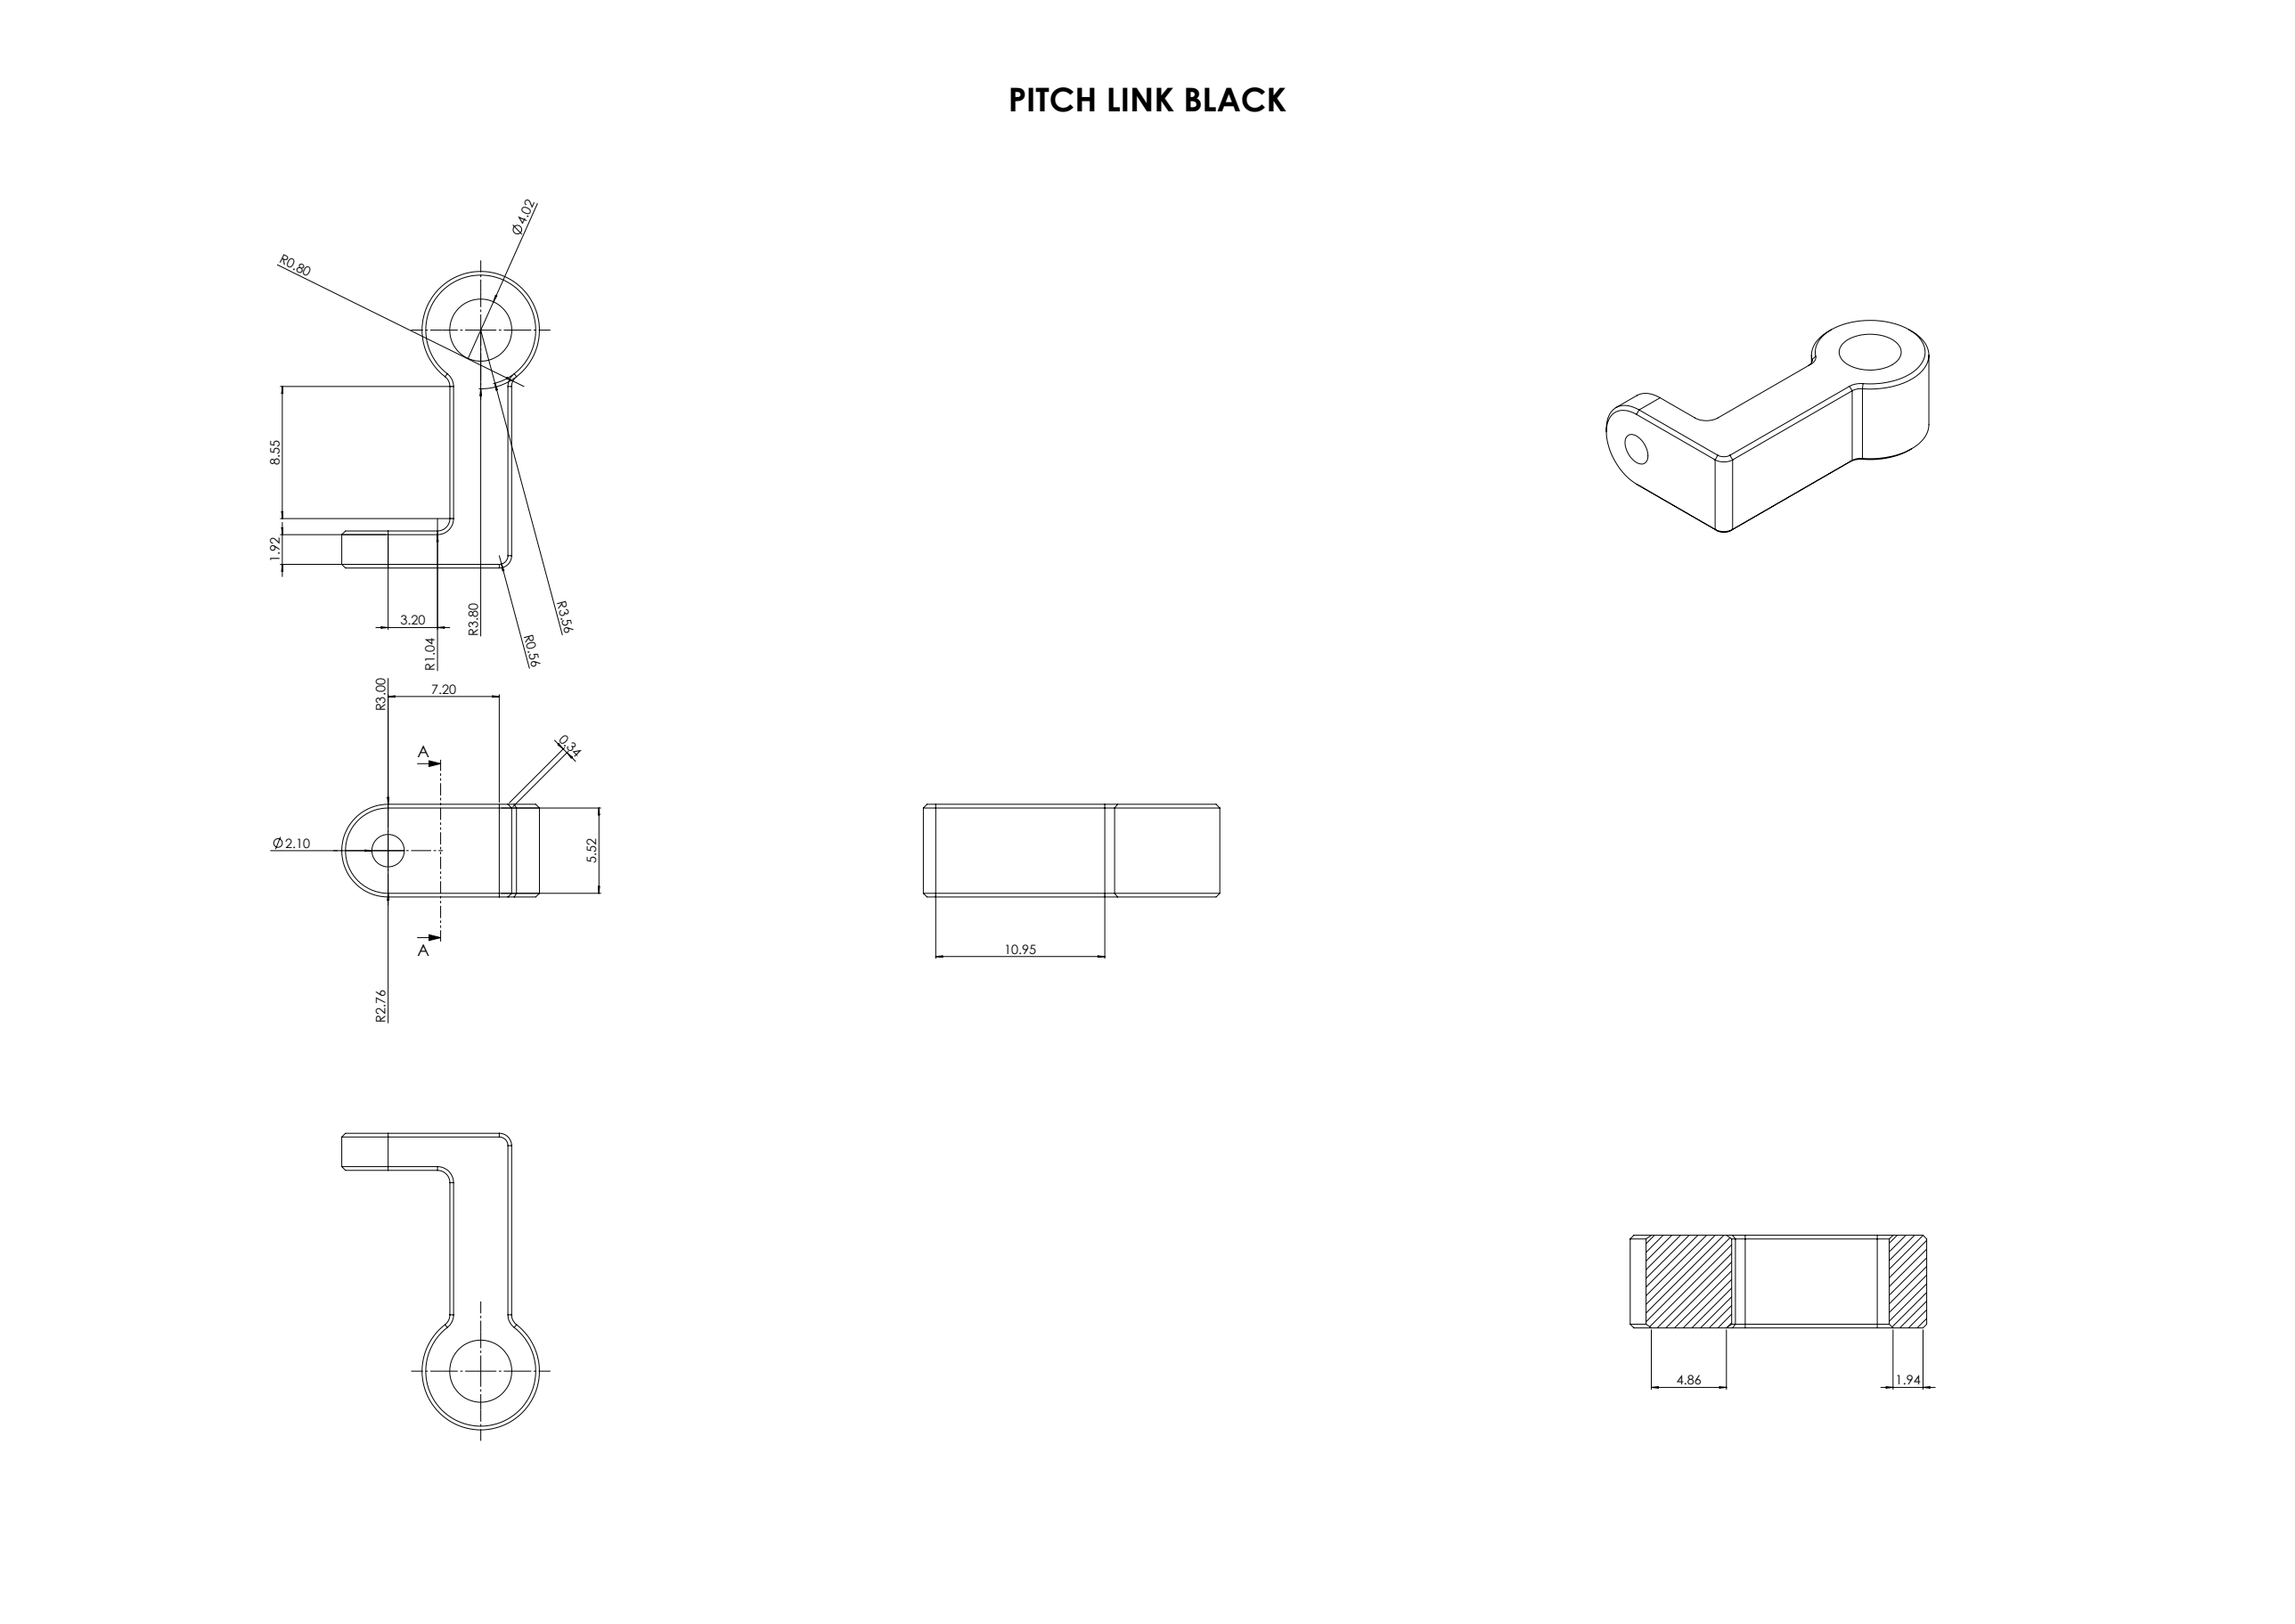
ISO-10303-21;
HEADER;
/* Generated by software containing ST-Developer
 * from STEP Tools, Inc. (www.steptools.com) 
 */

FILE_DESCRIPTION(
/* description */ (''),
/* implementation_level */ '2;1');

FILE_NAME(
/* name */ '07_Pitch_Link_Black.step',
/* time_stamp */ '2026-10-25T01:35:35-07:00',
/* author */ (''),
/* organization */ (''),
/* preprocessor_version */ 'ST-DEVELOPER v20.2',
/* originating_system */ 'Autodesk Translation Framework v15.15.0.0',
/* authorisation */ '');

FILE_SCHEMA (('AUTOMOTIVE_DESIGN { 1 0 10303 214 3 1 1 }'));
ENDSEC;

DATA;
#10=MECHANICAL_DESIGN_GEOMETRIC_PRESENTATION_REPRESENTATION('',(#268),#11430);
#244=SHAPE_REPRESENTATION_RELATIONSHIP('SRR','None',#11487,#256);
#256=ADVANCED_BREP_SHAPE_REPRESENTATION('',(#280),#11426);
#268=STYLED_ITEM('',(#11623),#280);
#280=MANIFOLD_SOLID_BREP('Body1',#4469);
#312=FACE_BOUND('',#1015,.T.);
#313=FACE_BOUND('',#1022,.T.);
#314=FACE_BOUND('',#1029,.T.);
#315=FACE_BOUND('',#1031,.T.);
#395=PLANE('',#4915);
#396=PLANE('',#4919);
#397=PLANE('',#4923);
#398=PLANE('',#4927);
#399=PLANE('',#4937);
#400=PLANE('',#4941);
#401=PLANE('',#4945);
#402=PLANE('',#4949);
#403=PLANE('',#4959);
#404=PLANE('',#4965);
#405=PLANE('',#4966);
#406=PLANE('',#4969);
#407=PLANE('',#4975);
#408=PLANE('',#4976);
#486=CYLINDRICAL_SURFACE('',#4961,0.8);
#487=CYLINDRICAL_SURFACE('',#4962,3.8);
#488=CYLINDRICAL_SURFACE('',#4963,0.8);
#489=CYLINDRICAL_SURFACE('',#4964,0.8);
#490=CYLINDRICAL_SURFACE('',#4968,3.);
#491=CYLINDRICAL_SURFACE('',#4970,0.8);
#492=CYLINDRICAL_SURFACE('',#4971,2.01);
#493=CYLINDRICAL_SURFACE('',#4973,1.05);
#698=FACE_OUTER_BOUND('',#994,.T.);
#699=FACE_OUTER_BOUND('',#995,.T.);
#700=FACE_OUTER_BOUND('',#996,.T.);
#701=FACE_OUTER_BOUND('',#997,.T.);
#702=FACE_OUTER_BOUND('',#998,.T.);
#703=FACE_OUTER_BOUND('',#999,.T.);
#704=FACE_OUTER_BOUND('',#1000,.T.);
#705=FACE_OUTER_BOUND('',#1001,.T.);
#706=FACE_OUTER_BOUND('',#1002,.T.);
#707=FACE_OUTER_BOUND('',#1003,.T.);
#708=FACE_OUTER_BOUND('',#1004,.T.);
#709=FACE_OUTER_BOUND('',#1005,.T.);
#710=FACE_OUTER_BOUND('',#1006,.T.);
#711=FACE_OUTER_BOUND('',#1007,.T.);
#712=FACE_OUTER_BOUND('',#1008,.T.);
#713=FACE_OUTER_BOUND('',#1009,.T.);
#714=FACE_OUTER_BOUND('',#1010,.T.);
#715=FACE_OUTER_BOUND('',#1011,.T.);
#716=FACE_OUTER_BOUND('',#1012,.T.);
#717=FACE_OUTER_BOUND('',#1013,.T.);
#718=FACE_OUTER_BOUND('',#1014,.T.);
#719=FACE_OUTER_BOUND('',#1016,.T.);
#720=FACE_OUTER_BOUND('',#1017,.T.);
#721=FACE_OUTER_BOUND('',#1018,.T.);
#722=FACE_OUTER_BOUND('',#1019,.T.);
#723=FACE_OUTER_BOUND('',#1020,.T.);
#724=FACE_OUTER_BOUND('',#1021,.T.);
#725=FACE_OUTER_BOUND('',#1023,.T.);
#726=FACE_OUTER_BOUND('',#1024,.T.);
#727=FACE_OUTER_BOUND('',#1025,.T.);
#728=FACE_OUTER_BOUND('',#1026,.T.);
#729=FACE_OUTER_BOUND('',#1027,.T.);
#730=FACE_OUTER_BOUND('',#1028,.T.);
#731=FACE_OUTER_BOUND('',#1030,.T.);
#994=EDGE_LOOP('',(#3675,#3676,#3677,#3678));
#995=EDGE_LOOP('',(#3679,#3680,#3681,#3682));
#996=EDGE_LOOP('',(#3683,#3684,#3685,#3686));
#997=EDGE_LOOP('',(#3687,#3688,#3689,#3690));
#998=EDGE_LOOP('',(#3691,#3692,#3693,#3694));
#999=EDGE_LOOP('',(#3695,#3696,#3697,#3698));
#1000=EDGE_LOOP('',(#3699,#3700,#3701,#3702));
#1001=EDGE_LOOP('',(#3703,#3704,#3705,#3706));
#1002=EDGE_LOOP('',(#3707,#3708,#3709,#3710));
#1003=EDGE_LOOP('',(#3711,#3712,#3713,#3714));
#1004=EDGE_LOOP('',(#3715,#3716,#3717,#3718));
#1005=EDGE_LOOP('',(#3719,#3720,#3721,#3722));
#1006=EDGE_LOOP('',(#3723,#3724,#3725,#3726));
#1007=EDGE_LOOP('',(#3727,#3728,#3729,#3730));
#1008=EDGE_LOOP('',(#3731,#3732,#3733,#3734));
#1009=EDGE_LOOP('',(#3735,#3736,#3737,#3738));
#1010=EDGE_LOOP('',(#3739,#3740,#3741,#3742));
#1011=EDGE_LOOP('',(#3743,#3744,#3745,#3746));
#1012=EDGE_LOOP('',(#3747,#3748,#3749,#3750));
#1013=EDGE_LOOP('',(#3751,#3752,#3753,#3754));
#1014=EDGE_LOOP('',(#3755,#3756,#3757,#3758));
#1015=EDGE_LOOP('',(#3759));
#1016=EDGE_LOOP('',(#3760,#3761,#3762,#3763));
#1017=EDGE_LOOP('',(#3764,#3765,#3766,#3767));
#1018=EDGE_LOOP('',(#3768,#3769,#3770,#3771));
#1019=EDGE_LOOP('',(#3772,#3773,#3774,#3775));
#1020=EDGE_LOOP('',(#3776,#3777,#3778,#3779));
#1021=EDGE_LOOP('',(#3780,#3781,#3782,#3783,#3784,#3785,#3786,#3787,#3788,
#3789));
#1022=EDGE_LOOP('',(#3790));
#1023=EDGE_LOOP('',(#3791,#3792,#3793,#3794));
#1024=EDGE_LOOP('',(#3795,#3796,#3797,#3798));
#1025=EDGE_LOOP('',(#3799,#3800,#3801,#3802));
#1026=EDGE_LOOP('',(#3803,#3804,#3805,#3806));
#1027=EDGE_LOOP('',(#3807,#3808,#3809,#3810));
#1028=EDGE_LOOP('',(#3811,#3812,#3813,#3814,#3815,#3816,#3817,#3818,#3819,
#3820));
#1029=EDGE_LOOP('',(#3821));
#1030=EDGE_LOOP('',(#3822,#3823,#3824,#3825));
#1031=EDGE_LOOP('',(#3826));
#1271=LINE('',#9219,#1561);
#1272=LINE('',#9221,#1562);
#1273=LINE('',#9223,#1563);
#1274=LINE('',#9224,#1564);
#1275=LINE('',#9229,#1565);
#1276=LINE('',#9233,#1566);
#1277=LINE('',#9235,#1567);
#1278=LINE('',#9236,#1568);
#1279=LINE('',#9241,#1569);
#1280=LINE('',#9245,#1570);
#1281=LINE('',#9247,#1571);
#1282=LINE('',#9248,#1572);
#1283=LINE('',#9253,#1573);
#1284=LINE('',#9258,#1574);
#1285=LINE('',#9259,#1575);
#1286=LINE('',#9260,#1576);
#1287=LINE('',#9265,#1577);
#1288=LINE('',#9270,#1578);
#1289=LINE('',#9277,#1579);
#1290=LINE('',#9282,#1580);
#1291=LINE('',#9283,#1581);
#1292=LINE('',#9284,#1582);
#1293=LINE('',#9289,#1583);
#1294=LINE('',#9294,#1584);
#1295=LINE('',#9295,#1585);
#1296=LINE('',#9296,#1586);
#1297=LINE('',#9300,#1587);
#1298=LINE('',#9306,#1588);
#1299=LINE('',#9307,#1589);
#1300=LINE('',#9308,#1590);
#1301=LINE('',#9313,#1591);
#1302=LINE('',#9317,#1592);
#1303=LINE('',#9319,#1593);
#1304=LINE('',#9320,#1594);
#1305=LINE('',#9325,#1595);
#1306=LINE('',#9331,#1596);
#1307=LINE('',#9337,#1597);
#1308=LINE('',#9341,#1598);
#1309=LINE('',#9342,#1599);
#1310=LINE('',#9344,#1600);
#1311=LINE('',#9346,#1601);
#1312=LINE('',#9348,#1602);
#1313=LINE('',#9351,#1603);
#1314=LINE('',#9355,#1604);
#1315=LINE('',#9357,#1605);
#1316=LINE('',#9359,#1606);
#1317=LINE('',#9362,#1607);
#1318=LINE('',#9366,#1608);
#1561=VECTOR('',#5873,10.);
#1562=VECTOR('',#5874,10.);
#1563=VECTOR('',#5875,10.);
#1564=VECTOR('',#5876,10.);
#1565=VECTOR('',#5881,10.);
#1566=VECTOR('',#5886,10.);
#1567=VECTOR('',#5887,10.);
#1568=VECTOR('',#5888,10.);
#1569=VECTOR('',#5893,10.);
#1570=VECTOR('',#5898,10.);
#1571=VECTOR('',#5899,10.);
#1572=VECTOR('',#5900,10.);
#1573=VECTOR('',#5905,10.);
#1574=VECTOR('',#5910,10.);
#1575=VECTOR('',#5911,10.);
#1576=VECTOR('',#5912,10.);
#1577=VECTOR('',#5917,10.);
#1578=VECTOR('',#5922,10.);
#1579=VECTOR('',#5931,10.);
#1580=VECTOR('',#5936,10.);
#1581=VECTOR('',#5937,10.);
#1582=VECTOR('',#5938,10.);
#1583=VECTOR('',#5943,10.);
#1584=VECTOR('',#5948,10.);
#1585=VECTOR('',#5949,10.);
#1586=VECTOR('',#5950,10.);
#1587=VECTOR('',#5953,10.);
#1588=VECTOR('',#5960,10.);
#1589=VECTOR('',#5961,10.);
#1590=VECTOR('',#5962,10.);
#1591=VECTOR('',#5967,10.);
#1592=VECTOR('',#5972,10.);
#1593=VECTOR('',#5973,10.);
#1594=VECTOR('',#5974,10.);
#1595=VECTOR('',#5979,10.);
#1596=VECTOR('',#5986,10.);
#1597=VECTOR('',#5997,10.);
#1598=VECTOR('',#6002,10.);
#1599=VECTOR('',#6003,10.);
#1600=VECTOR('',#6006,10.);
#1601=VECTOR('',#6009,10.);
#1602=VECTOR('',#6012,10.);
#1603=VECTOR('',#6017,10.);
#1604=VECTOR('',#6022,10.);
#1605=VECTOR('',#6025,10.);
#1606=VECTOR('',#6028,10.);
#1607=VECTOR('',#6031,2.01);
#1608=VECTOR('',#6036,1.05);
#1812=CIRCLE('',#4917,0.8);
#1813=CIRCLE('',#4918,0.56);
#1814=CIRCLE('',#4921,2.76);
#1815=CIRCLE('',#4922,3.);
#1816=CIRCLE('',#4925,0.8);
#1817=CIRCLE('',#4926,0.56);
#1818=CIRCLE('',#4929,0.8);
#1819=CIRCLE('',#4930,1.04);
#1820=CIRCLE('',#4932,3.56);
#1821=CIRCLE('',#4933,3.8);
#1822=CIRCLE('',#4935,0.8);
#1823=CIRCLE('',#4936,1.04);
#1824=CIRCLE('',#4939,0.8);
#1825=CIRCLE('',#4940,1.04);
#1826=CIRCLE('',#4943,3.);
#1827=CIRCLE('',#4944,2.76);
#1828=CIRCLE('',#4947,0.8);
#1829=CIRCLE('',#4948,1.04);
#1830=CIRCLE('',#4951,0.8);
#1831=CIRCLE('',#4952,1.04);
#1832=CIRCLE('',#4954,3.8);
#1833=CIRCLE('',#4955,3.56);
#1834=CIRCLE('',#4957,0.8);
#1835=CIRCLE('',#4958,1.04);
#1836=CIRCLE('',#4960,1.05);
#1837=CIRCLE('',#4967,2.01);
#1838=CIRCLE('',#4972,2.01);
#1839=CIRCLE('',#4974,1.05);
#2115=VERTEX_POINT('',#9217);
#2116=VERTEX_POINT('',#9218);
#2117=VERTEX_POINT('',#9220);
#2118=VERTEX_POINT('',#9222);
#2119=VERTEX_POINT('',#9226);
#2120=VERTEX_POINT('',#9228);
#2121=VERTEX_POINT('',#9232);
#2122=VERTEX_POINT('',#9234);
#2123=VERTEX_POINT('',#9238);
#2124=VERTEX_POINT('',#9240);
#2125=VERTEX_POINT('',#9244);
#2126=VERTEX_POINT('',#9246);
#2127=VERTEX_POINT('',#9250);
#2128=VERTEX_POINT('',#9252);
#2129=VERTEX_POINT('',#9256);
#2130=VERTEX_POINT('',#9257);
#2131=VERTEX_POINT('',#9262);
#2132=VERTEX_POINT('',#9264);
#2133=VERTEX_POINT('',#9268);
#2134=VERTEX_POINT('',#9269);
#2135=VERTEX_POINT('',#9274);
#2136=VERTEX_POINT('',#9276);
#2137=VERTEX_POINT('',#9280);
#2138=VERTEX_POINT('',#9281);
#2139=VERTEX_POINT('',#9286);
#2140=VERTEX_POINT('',#9288);
#2141=VERTEX_POINT('',#9292);
#2142=VERTEX_POINT('',#9293);
#2143=VERTEX_POINT('',#9298);
#2144=VERTEX_POINT('',#9299);
#2145=VERTEX_POINT('',#9304);
#2146=VERTEX_POINT('',#9305);
#2147=VERTEX_POINT('',#9310);
#2148=VERTEX_POINT('',#9312);
#2149=VERTEX_POINT('',#9316);
#2150=VERTEX_POINT('',#9318);
#2151=VERTEX_POINT('',#9322);
#2152=VERTEX_POINT('',#9324);
#2153=VERTEX_POINT('',#9328);
#2154=VERTEX_POINT('',#9330);
#2155=VERTEX_POINT('',#9338);
#2156=VERTEX_POINT('',#9352);
#2157=VERTEX_POINT('',#9361);
#2158=VERTEX_POINT('',#9365);
#2655=EDGE_CURVE('',#2115,#2116,#1271,.T.);
#2656=EDGE_CURVE('',#2116,#2117,#1272,.T.);
#2657=EDGE_CURVE('',#2117,#2118,#1273,.T.);
#2658=EDGE_CURVE('',#2118,#2115,#1274,.T.);
#2659=EDGE_CURVE('',#2115,#2119,#1812,.T.);
#2660=EDGE_CURVE('',#2119,#2120,#1275,.T.);
#2661=EDGE_CURVE('',#2120,#2116,#1813,.T.);
#2662=EDGE_CURVE('',#2119,#2121,#1276,.T.);
#2663=EDGE_CURVE('',#2121,#2122,#1277,.T.);
#2664=EDGE_CURVE('',#2122,#2120,#1278,.T.);
#2665=EDGE_CURVE('',#2121,#2123,#1814,.T.);
#2666=EDGE_CURVE('',#2123,#2124,#1279,.T.);
#2667=EDGE_CURVE('',#2124,#2122,#1815,.T.);
#2668=EDGE_CURVE('',#2123,#2125,#1280,.T.);
#2669=EDGE_CURVE('',#2125,#2126,#1281,.T.);
#2670=EDGE_CURVE('',#2126,#2124,#1282,.T.);
#2671=EDGE_CURVE('',#2125,#2127,#1816,.T.);
#2672=EDGE_CURVE('',#2127,#2128,#1283,.T.);
#2673=EDGE_CURVE('',#2128,#2126,#1817,.T.);
#2674=EDGE_CURVE('',#2129,#2130,#1284,.T.);
#2675=EDGE_CURVE('',#2130,#2128,#1285,.T.);
#2676=EDGE_CURVE('',#2127,#2129,#1286,.T.);
#2677=EDGE_CURVE('',#2129,#2131,#1818,.T.);
#2678=EDGE_CURVE('',#2131,#2132,#1287,.T.);
#2679=EDGE_CURVE('',#2132,#2130,#1819,.T.);
#2680=EDGE_CURVE('',#2133,#2134,#1288,.T.);
#2681=EDGE_CURVE('',#2134,#2132,#1820,.T.);
#2682=EDGE_CURVE('',#2131,#2133,#1821,.T.);
#2683=EDGE_CURVE('',#2133,#2135,#1822,.T.);
#2684=EDGE_CURVE('',#2135,#2136,#1289,.T.);
#2685=EDGE_CURVE('',#2136,#2134,#1823,.T.);
#2686=EDGE_CURVE('',#2137,#2138,#1290,.T.);
#2687=EDGE_CURVE('',#2138,#2136,#1291,.T.);
#2688=EDGE_CURVE('',#2135,#2137,#1292,.T.);
#2689=EDGE_CURVE('',#2137,#2139,#1824,.T.);
#2690=EDGE_CURVE('',#2139,#2140,#1293,.T.);
#2691=EDGE_CURVE('',#2140,#2138,#1825,.T.);
#2692=EDGE_CURVE('',#2141,#2142,#1294,.T.);
#2693=EDGE_CURVE('',#2142,#2140,#1295,.T.);
#2694=EDGE_CURVE('',#2139,#2141,#1296,.T.);
#2695=EDGE_CURVE('',#2143,#2144,#1297,.T.);
#2696=EDGE_CURVE('',#2144,#2142,#1826,.T.);
#2697=EDGE_CURVE('',#2141,#2143,#1827,.T.);
#2698=EDGE_CURVE('',#2145,#2146,#1298,.T.);
#2699=EDGE_CURVE('',#2146,#2144,#1299,.T.);
#2700=EDGE_CURVE('',#2143,#2145,#1300,.T.);
#2701=EDGE_CURVE('',#2145,#2147,#1828,.T.);
#2702=EDGE_CURVE('',#2147,#2148,#1301,.T.);
#2703=EDGE_CURVE('',#2148,#2146,#1829,.T.);
#2704=EDGE_CURVE('',#2147,#2149,#1302,.T.);
#2705=EDGE_CURVE('',#2149,#2150,#1303,.T.);
#2706=EDGE_CURVE('',#2150,#2148,#1304,.T.);
#2707=EDGE_CURVE('',#2149,#2151,#1830,.T.);
#2708=EDGE_CURVE('',#2151,#2152,#1305,.T.);
#2709=EDGE_CURVE('',#2152,#2150,#1831,.T.);
#2710=EDGE_CURVE('',#2151,#2153,#1832,.T.);
#2711=EDGE_CURVE('',#2153,#2154,#1306,.T.);
#2712=EDGE_CURVE('',#2154,#2152,#1833,.T.);
#2713=EDGE_CURVE('',#2153,#2118,#1834,.T.);
#2714=EDGE_CURVE('',#2117,#2154,#1835,.T.);
#2715=EDGE_CURVE('',#2125,#2119,#1307,.T.);
#2716=EDGE_CURVE('',#2155,#2155,#1836,.T.);
#2717=EDGE_CURVE('',#2133,#2151,#1308,.T.);
#2718=EDGE_CURVE('',#2149,#2135,#1309,.T.);
#2719=EDGE_CURVE('',#2153,#2131,#1310,.T.);
#2720=EDGE_CURVE('',#2115,#2127,#1311,.T.);
#2721=EDGE_CURVE('',#2129,#2118,#1312,.T.);
#2722=EDGE_CURVE('',#2144,#2122,#1313,.T.);
#2723=EDGE_CURVE('',#2156,#2156,#1837,.T.);
#2724=EDGE_CURVE('',#2142,#2124,#1314,.T.);
#2725=EDGE_CURVE('',#2137,#2147,#1315,.T.);
#2726=EDGE_CURVE('',#2145,#2139,#1316,.T.);
#2727=EDGE_CURVE('',#2156,#2157,#1317,.T.);
#2728=EDGE_CURVE('',#2157,#2157,#1838,.T.);
#2729=EDGE_CURVE('',#2155,#2158,#1318,.T.);
#2730=EDGE_CURVE('',#2158,#2158,#1839,.T.);
#3675=ORIENTED_EDGE('',*,*,#2655,.T.);
#3676=ORIENTED_EDGE('',*,*,#2656,.T.);
#3677=ORIENTED_EDGE('',*,*,#2657,.T.);
#3678=ORIENTED_EDGE('',*,*,#2658,.T.);
#3679=ORIENTED_EDGE('',*,*,#2655,.F.);
#3680=ORIENTED_EDGE('',*,*,#2659,.T.);
#3681=ORIENTED_EDGE('',*,*,#2660,.T.);
#3682=ORIENTED_EDGE('',*,*,#2661,.T.);
#3683=ORIENTED_EDGE('',*,*,#2660,.F.);
#3684=ORIENTED_EDGE('',*,*,#2662,.T.);
#3685=ORIENTED_EDGE('',*,*,#2663,.T.);
#3686=ORIENTED_EDGE('',*,*,#2664,.T.);
#3687=ORIENTED_EDGE('',*,*,#2663,.F.);
#3688=ORIENTED_EDGE('',*,*,#2665,.T.);
#3689=ORIENTED_EDGE('',*,*,#2666,.T.);
#3690=ORIENTED_EDGE('',*,*,#2667,.T.);
#3691=ORIENTED_EDGE('',*,*,#2666,.F.);
#3692=ORIENTED_EDGE('',*,*,#2668,.T.);
#3693=ORIENTED_EDGE('',*,*,#2669,.T.);
#3694=ORIENTED_EDGE('',*,*,#2670,.T.);
#3695=ORIENTED_EDGE('',*,*,#2669,.F.);
#3696=ORIENTED_EDGE('',*,*,#2671,.T.);
#3697=ORIENTED_EDGE('',*,*,#2672,.T.);
#3698=ORIENTED_EDGE('',*,*,#2673,.T.);
#3699=ORIENTED_EDGE('',*,*,#2674,.T.);
#3700=ORIENTED_EDGE('',*,*,#2675,.T.);
#3701=ORIENTED_EDGE('',*,*,#2672,.F.);
#3702=ORIENTED_EDGE('',*,*,#2676,.T.);
#3703=ORIENTED_EDGE('',*,*,#2674,.F.);
#3704=ORIENTED_EDGE('',*,*,#2677,.T.);
#3705=ORIENTED_EDGE('',*,*,#2678,.T.);
#3706=ORIENTED_EDGE('',*,*,#2679,.T.);
#3707=ORIENTED_EDGE('',*,*,#2680,.T.);
#3708=ORIENTED_EDGE('',*,*,#2681,.T.);
#3709=ORIENTED_EDGE('',*,*,#2678,.F.);
#3710=ORIENTED_EDGE('',*,*,#2682,.T.);
#3711=ORIENTED_EDGE('',*,*,#2680,.F.);
#3712=ORIENTED_EDGE('',*,*,#2683,.T.);
#3713=ORIENTED_EDGE('',*,*,#2684,.T.);
#3714=ORIENTED_EDGE('',*,*,#2685,.T.);
#3715=ORIENTED_EDGE('',*,*,#2686,.T.);
#3716=ORIENTED_EDGE('',*,*,#2687,.T.);
#3717=ORIENTED_EDGE('',*,*,#2684,.F.);
#3718=ORIENTED_EDGE('',*,*,#2688,.T.);
#3719=ORIENTED_EDGE('',*,*,#2686,.F.);
#3720=ORIENTED_EDGE('',*,*,#2689,.T.);
#3721=ORIENTED_EDGE('',*,*,#2690,.T.);
#3722=ORIENTED_EDGE('',*,*,#2691,.T.);
#3723=ORIENTED_EDGE('',*,*,#2692,.T.);
#3724=ORIENTED_EDGE('',*,*,#2693,.T.);
#3725=ORIENTED_EDGE('',*,*,#2690,.F.);
#3726=ORIENTED_EDGE('',*,*,#2694,.T.);
#3727=ORIENTED_EDGE('',*,*,#2695,.T.);
#3728=ORIENTED_EDGE('',*,*,#2696,.T.);
#3729=ORIENTED_EDGE('',*,*,#2692,.F.);
#3730=ORIENTED_EDGE('',*,*,#2697,.T.);
#3731=ORIENTED_EDGE('',*,*,#2698,.T.);
#3732=ORIENTED_EDGE('',*,*,#2699,.T.);
#3733=ORIENTED_EDGE('',*,*,#2695,.F.);
#3734=ORIENTED_EDGE('',*,*,#2700,.T.);
#3735=ORIENTED_EDGE('',*,*,#2698,.F.);
#3736=ORIENTED_EDGE('',*,*,#2701,.T.);
#3737=ORIENTED_EDGE('',*,*,#2702,.T.);
#3738=ORIENTED_EDGE('',*,*,#2703,.T.);
#3739=ORIENTED_EDGE('',*,*,#2702,.F.);
#3740=ORIENTED_EDGE('',*,*,#2704,.T.);
#3741=ORIENTED_EDGE('',*,*,#2705,.T.);
#3742=ORIENTED_EDGE('',*,*,#2706,.T.);
#3743=ORIENTED_EDGE('',*,*,#2705,.F.);
#3744=ORIENTED_EDGE('',*,*,#2707,.T.);
#3745=ORIENTED_EDGE('',*,*,#2708,.T.);
#3746=ORIENTED_EDGE('',*,*,#2709,.T.);
#3747=ORIENTED_EDGE('',*,*,#2708,.F.);
#3748=ORIENTED_EDGE('',*,*,#2710,.T.);
#3749=ORIENTED_EDGE('',*,*,#2711,.T.);
#3750=ORIENTED_EDGE('',*,*,#2712,.T.);
#3751=ORIENTED_EDGE('',*,*,#2711,.F.);
#3752=ORIENTED_EDGE('',*,*,#2713,.T.);
#3753=ORIENTED_EDGE('',*,*,#2657,.F.);
#3754=ORIENTED_EDGE('',*,*,#2714,.T.);
#3755=ORIENTED_EDGE('',*,*,#2668,.F.);
#3756=ORIENTED_EDGE('',*,*,#2665,.F.);
#3757=ORIENTED_EDGE('',*,*,#2662,.F.);
#3758=ORIENTED_EDGE('',*,*,#2715,.F.);
#3759=ORIENTED_EDGE('',*,*,#2716,.T.);
#3760=ORIENTED_EDGE('',*,*,#2683,.F.);
#3761=ORIENTED_EDGE('',*,*,#2717,.T.);
#3762=ORIENTED_EDGE('',*,*,#2707,.F.);
#3763=ORIENTED_EDGE('',*,*,#2718,.T.);
#3764=ORIENTED_EDGE('',*,*,#2682,.F.);
#3765=ORIENTED_EDGE('',*,*,#2719,.F.);
#3766=ORIENTED_EDGE('',*,*,#2710,.F.);
#3767=ORIENTED_EDGE('',*,*,#2717,.F.);
#3768=ORIENTED_EDGE('',*,*,#2671,.F.);
#3769=ORIENTED_EDGE('',*,*,#2715,.T.);
#3770=ORIENTED_EDGE('',*,*,#2659,.F.);
#3771=ORIENTED_EDGE('',*,*,#2720,.T.);
#3772=ORIENTED_EDGE('',*,*,#2677,.F.);
#3773=ORIENTED_EDGE('',*,*,#2721,.T.);
#3774=ORIENTED_EDGE('',*,*,#2713,.F.);
#3775=ORIENTED_EDGE('',*,*,#2719,.T.);
#3776=ORIENTED_EDGE('',*,*,#2676,.F.);
#3777=ORIENTED_EDGE('',*,*,#2720,.F.);
#3778=ORIENTED_EDGE('',*,*,#2658,.F.);
#3779=ORIENTED_EDGE('',*,*,#2721,.F.);
#3780=ORIENTED_EDGE('',*,*,#2699,.F.);
#3781=ORIENTED_EDGE('',*,*,#2703,.F.);
#3782=ORIENTED_EDGE('',*,*,#2706,.F.);
#3783=ORIENTED_EDGE('',*,*,#2709,.F.);
#3784=ORIENTED_EDGE('',*,*,#2712,.F.);
#3785=ORIENTED_EDGE('',*,*,#2714,.F.);
#3786=ORIENTED_EDGE('',*,*,#2656,.F.);
#3787=ORIENTED_EDGE('',*,*,#2661,.F.);
#3788=ORIENTED_EDGE('',*,*,#2664,.F.);
#3789=ORIENTED_EDGE('',*,*,#2722,.F.);
#3790=ORIENTED_EDGE('',*,*,#2723,.T.);
#3791=ORIENTED_EDGE('',*,*,#2696,.F.);
#3792=ORIENTED_EDGE('',*,*,#2722,.T.);
#3793=ORIENTED_EDGE('',*,*,#2667,.F.);
#3794=ORIENTED_EDGE('',*,*,#2724,.F.);
#3795=ORIENTED_EDGE('',*,*,#2688,.F.);
#3796=ORIENTED_EDGE('',*,*,#2718,.F.);
#3797=ORIENTED_EDGE('',*,*,#2704,.F.);
#3798=ORIENTED_EDGE('',*,*,#2725,.F.);
#3799=ORIENTED_EDGE('',*,*,#2689,.F.);
#3800=ORIENTED_EDGE('',*,*,#2725,.T.);
#3801=ORIENTED_EDGE('',*,*,#2701,.F.);
#3802=ORIENTED_EDGE('',*,*,#2726,.T.);
#3803=ORIENTED_EDGE('',*,*,#2723,.F.);
#3804=ORIENTED_EDGE('',*,*,#2727,.T.);
#3805=ORIENTED_EDGE('',*,*,#2728,.F.);
#3806=ORIENTED_EDGE('',*,*,#2727,.F.);
#3807=ORIENTED_EDGE('',*,*,#2716,.F.);
#3808=ORIENTED_EDGE('',*,*,#2729,.T.);
#3809=ORIENTED_EDGE('',*,*,#2730,.F.);
#3810=ORIENTED_EDGE('',*,*,#2729,.F.);
#3811=ORIENTED_EDGE('',*,*,#2693,.F.);
#3812=ORIENTED_EDGE('',*,*,#2724,.T.);
#3813=ORIENTED_EDGE('',*,*,#2670,.F.);
#3814=ORIENTED_EDGE('',*,*,#2673,.F.);
#3815=ORIENTED_EDGE('',*,*,#2675,.F.);
#3816=ORIENTED_EDGE('',*,*,#2679,.F.);
#3817=ORIENTED_EDGE('',*,*,#2681,.F.);
#3818=ORIENTED_EDGE('',*,*,#2685,.F.);
#3819=ORIENTED_EDGE('',*,*,#2687,.F.);
#3820=ORIENTED_EDGE('',*,*,#2691,.F.);
#3821=ORIENTED_EDGE('',*,*,#2728,.T.);
#3822=ORIENTED_EDGE('',*,*,#2694,.F.);
#3823=ORIENTED_EDGE('',*,*,#2726,.F.);
#3824=ORIENTED_EDGE('',*,*,#2700,.F.);
#3825=ORIENTED_EDGE('',*,*,#2697,.F.);
#3826=ORIENTED_EDGE('',*,*,#2730,.T.);
#4175=CONICAL_SURFACE('',#4916,0.68,0.785398163397448);
#4176=CONICAL_SURFACE('',#4920,2.88,0.785398163397448);
#4177=CONICAL_SURFACE('',#4924,0.68,0.785398163397447);
#4178=CONICAL_SURFACE('',#4928,0.92,0.785398163397448);
#4179=CONICAL_SURFACE('',#4931,3.68,0.785398163397451);
#4180=CONICAL_SURFACE('',#4934,0.92,0.785398163397448);
#4181=CONICAL_SURFACE('',#4938,0.92,0.785398163397445);
#4182=CONICAL_SURFACE('',#4942,2.88,0.785398163397448);
#4183=CONICAL_SURFACE('',#4946,0.92,0.785398163397446);
#4184=CONICAL_SURFACE('',#4950,0.92,0.785398163397448);
#4185=CONICAL_SURFACE('',#4953,3.68,0.785398163397448);
#4186=CONICAL_SURFACE('',#4956,0.92,0.785398163397448);
#4365=ADVANCED_FACE('',(#698),#395,.T.);
#4366=ADVANCED_FACE('',(#699),#4175,.T.);
#4367=ADVANCED_FACE('',(#700),#396,.T.);
#4368=ADVANCED_FACE('',(#701),#4176,.T.);
#4369=ADVANCED_FACE('',(#702),#397,.T.);
#4370=ADVANCED_FACE('',(#703),#4177,.T.);
#4371=ADVANCED_FACE('',(#704),#398,.T.);
#4372=ADVANCED_FACE('',(#705),#4178,.F.);
#4373=ADVANCED_FACE('',(#706),#4179,.T.);
#4374=ADVANCED_FACE('',(#707),#4180,.F.);
#4375=ADVANCED_FACE('',(#708),#399,.T.);
#4376=ADVANCED_FACE('',(#709),#4181,.F.);
#4377=ADVANCED_FACE('',(#710),#400,.T.);
#4378=ADVANCED_FACE('',(#711),#4182,.T.);
#4379=ADVANCED_FACE('',(#712),#401,.T.);
#4380=ADVANCED_FACE('',(#713),#4183,.F.);
#4381=ADVANCED_FACE('',(#714),#402,.T.);
#4382=ADVANCED_FACE('',(#715),#4184,.F.);
#4383=ADVANCED_FACE('',(#716),#4185,.T.);
#4384=ADVANCED_FACE('',(#717),#4186,.F.);
#4385=ADVANCED_FACE('',(#718,#312),#403,.T.);
#4386=ADVANCED_FACE('',(#719),#486,.F.);
#4387=ADVANCED_FACE('',(#720),#487,.T.);
#4388=ADVANCED_FACE('',(#721),#488,.T.);
#4389=ADVANCED_FACE('',(#722),#489,.F.);
#4390=ADVANCED_FACE('',(#723),#404,.T.);
#4391=ADVANCED_FACE('',(#724,#313),#405,.T.);
#4392=ADVANCED_FACE('',(#725),#490,.T.);
#4393=ADVANCED_FACE('',(#726),#406,.T.);
#4394=ADVANCED_FACE('',(#727),#491,.F.);
#4395=ADVANCED_FACE('',(#728),#492,.F.);
#4396=ADVANCED_FACE('',(#729),#493,.F.);
#4397=ADVANCED_FACE('',(#730,#314),#407,.T.);
#4398=ADVANCED_FACE('',(#731,#315),#408,.F.);
#4469=CLOSED_SHELL('',(#4365,#4366,#4367,#4368,#4369,#4370,#4371,#4372,
#4373,#4374,#4375,#4376,#4377,#4378,#4379,#4380,#4381,#4382,#4383,#4384,
#4385,#4386,#4387,#4388,#4389,#4390,#4391,#4392,#4393,#4394,#4395,#4396,
#4397,#4398));
#4914=AXIS2_PLACEMENT_3D('',#9215,#5869,#5870);
#4915=AXIS2_PLACEMENT_3D('',#9216,#5871,#5872);
#4916=AXIS2_PLACEMENT_3D('',#9225,#5877,#5878);
#4917=AXIS2_PLACEMENT_3D('',#9227,#5879,#5880);
#4918=AXIS2_PLACEMENT_3D('',#9230,#5882,#5883);
#4919=AXIS2_PLACEMENT_3D('',#9231,#5884,#5885);
#4920=AXIS2_PLACEMENT_3D('',#9237,#5889,#5890);
#4921=AXIS2_PLACEMENT_3D('',#9239,#5891,#5892);
#4922=AXIS2_PLACEMENT_3D('',#9242,#5894,#5895);
#4923=AXIS2_PLACEMENT_3D('',#9243,#5896,#5897);
#4924=AXIS2_PLACEMENT_3D('',#9249,#5901,#5902);
#4925=AXIS2_PLACEMENT_3D('',#9251,#5903,#5904);
#4926=AXIS2_PLACEMENT_3D('',#9254,#5906,#5907);
#4927=AXIS2_PLACEMENT_3D('',#9255,#5908,#5909);
#4928=AXIS2_PLACEMENT_3D('',#9261,#5913,#5914);
#4929=AXIS2_PLACEMENT_3D('',#9263,#5915,#5916);
#4930=AXIS2_PLACEMENT_3D('',#9266,#5918,#5919);
#4931=AXIS2_PLACEMENT_3D('',#9267,#5920,#5921);
#4932=AXIS2_PLACEMENT_3D('',#9271,#5923,#5924);
#4933=AXIS2_PLACEMENT_3D('',#9272,#5925,#5926);
#4934=AXIS2_PLACEMENT_3D('',#9273,#5927,#5928);
#4935=AXIS2_PLACEMENT_3D('',#9275,#5929,#5930);
#4936=AXIS2_PLACEMENT_3D('',#9278,#5932,#5933);
#4937=AXIS2_PLACEMENT_3D('',#9279,#5934,#5935);
#4938=AXIS2_PLACEMENT_3D('',#9285,#5939,#5940);
#4939=AXIS2_PLACEMENT_3D('',#9287,#5941,#5942);
#4940=AXIS2_PLACEMENT_3D('',#9290,#5944,#5945);
#4941=AXIS2_PLACEMENT_3D('',#9291,#5946,#5947);
#4942=AXIS2_PLACEMENT_3D('',#9297,#5951,#5952);
#4943=AXIS2_PLACEMENT_3D('',#9301,#5954,#5955);
#4944=AXIS2_PLACEMENT_3D('',#9302,#5956,#5957);
#4945=AXIS2_PLACEMENT_3D('',#9303,#5958,#5959);
#4946=AXIS2_PLACEMENT_3D('',#9309,#5963,#5964);
#4947=AXIS2_PLACEMENT_3D('',#9311,#5965,#5966);
#4948=AXIS2_PLACEMENT_3D('',#9314,#5968,#5969);
#4949=AXIS2_PLACEMENT_3D('',#9315,#5970,#5971);
#4950=AXIS2_PLACEMENT_3D('',#9321,#5975,#5976);
#4951=AXIS2_PLACEMENT_3D('',#9323,#5977,#5978);
#4952=AXIS2_PLACEMENT_3D('',#9326,#5980,#5981);
#4953=AXIS2_PLACEMENT_3D('',#9327,#5982,#5983);
#4954=AXIS2_PLACEMENT_3D('',#9329,#5984,#5985);
#4955=AXIS2_PLACEMENT_3D('',#9332,#5987,#5988);
#4956=AXIS2_PLACEMENT_3D('',#9333,#5989,#5990);
#4957=AXIS2_PLACEMENT_3D('',#9334,#5991,#5992);
#4958=AXIS2_PLACEMENT_3D('',#9335,#5993,#5994);
#4959=AXIS2_PLACEMENT_3D('',#9336,#5995,#5996);
#4960=AXIS2_PLACEMENT_3D('',#9339,#5998,#5999);
#4961=AXIS2_PLACEMENT_3D('',#9340,#6000,#6001);
#4962=AXIS2_PLACEMENT_3D('',#9343,#6004,#6005);
#4963=AXIS2_PLACEMENT_3D('',#9345,#6007,#6008);
#4964=AXIS2_PLACEMENT_3D('',#9347,#6010,#6011);
#4965=AXIS2_PLACEMENT_3D('',#9349,#6013,#6014);
#4966=AXIS2_PLACEMENT_3D('',#9350,#6015,#6016);
#4967=AXIS2_PLACEMENT_3D('',#9353,#6018,#6019);
#4968=AXIS2_PLACEMENT_3D('',#9354,#6020,#6021);
#4969=AXIS2_PLACEMENT_3D('',#9356,#6023,#6024);
#4970=AXIS2_PLACEMENT_3D('',#9358,#6026,#6027);
#4971=AXIS2_PLACEMENT_3D('',#9360,#6029,#6030);
#4972=AXIS2_PLACEMENT_3D('',#9363,#6032,#6033);
#4973=AXIS2_PLACEMENT_3D('',#9364,#6034,#6035);
#4974=AXIS2_PLACEMENT_3D('',#9367,#6037,#6038);
#4975=AXIS2_PLACEMENT_3D('',#9368,#6039,#6040);
#4976=AXIS2_PLACEMENT_3D('',#9369,#6041,#6042);
#5869=DIRECTION('axis',(0.,0.,1.));
#5870=DIRECTION('refdir',(1.,0.,0.));
#5871=DIRECTION('center_axis',(0.707106781186548,-0.707106781186548,0.));
#5872=DIRECTION('ref_axis',(0.,0.,-1.));
#5873=DIRECTION('',(-0.707106781186547,-0.707106781186547,0.));
#5874=DIRECTION('',(0.,0.,-1.));
#5875=DIRECTION('',(0.707106781186547,0.707106781186547,0.));
#5876=DIRECTION('',(0.,0.,1.));
#5877=DIRECTION('center_axis',(0.,1.,0.));
#5878=DIRECTION('ref_axis',(0.707106781186547,0.,0.707106781186547));
#5879=DIRECTION('center_axis',(0.,-1.,0.));
#5880=DIRECTION('ref_axis',(0.707106781186548,0.,0.707106781186548));
#5881=DIRECTION('',(0.,-0.707106781186547,-0.707106781186547));
#5882=DIRECTION('center_axis',(0.,1.,0.));
#5883=DIRECTION('ref_axis',(0.707106781186547,0.,0.707106781186547));
#5884=DIRECTION('center_axis',(0.,-0.707106781186548,0.707106781186548));
#5885=DIRECTION('ref_axis',(1.,0.,0.));
#5886=DIRECTION('',(-1.,0.,0.));
#5887=DIRECTION('',(0.,-0.707106781186547,-0.707106781186547));
#5888=DIRECTION('',(1.,0.,0.));
#5889=DIRECTION('center_axis',(0.,0.,-1.));
#5890=DIRECTION('ref_axis',(-1.,0.,0.));
#5891=DIRECTION('center_axis',(0.,0.,-1.));
#5892=DIRECTION('ref_axis',(-1.,0.,0.));
#5893=DIRECTION('',(0.,0.707106781186547,-0.707106781186548));
#5894=DIRECTION('center_axis',(0.,0.,1.));
#5895=DIRECTION('ref_axis',(-1.,0.,0.));
#5896=DIRECTION('center_axis',(0.,0.707106781186548,0.707106781186548));
#5897=DIRECTION('ref_axis',(1.,0.,0.));
#5898=DIRECTION('',(1.,0.,0.));
#5899=DIRECTION('',(0.,0.707106781186548,-0.707106781186547));
#5900=DIRECTION('',(-1.,0.,0.));
#5901=DIRECTION('center_axis',(0.,-1.,0.));
#5902=DIRECTION('ref_axis',(0.707106781186547,0.,0.707106781186547));
#5903=DIRECTION('center_axis',(0.,1.,0.));
#5904=DIRECTION('ref_axis',(0.707106781186548,0.,0.707106781186548));
#5905=DIRECTION('',(-0.707106781186547,0.707106781186548,0.));
#5906=DIRECTION('center_axis',(0.,-1.,0.));
#5907=DIRECTION('ref_axis',(0.707106781186547,0.,0.707106781186547));
#5908=DIRECTION('center_axis',(0.707106781186546,0.707106781186549,0.));
#5909=DIRECTION('ref_axis',(0.,0.,-1.));
#5910=DIRECTION('',(-0.707106781186549,0.707106781186546,0.));
#5911=DIRECTION('',(0.,0.,1.));
#5912=DIRECTION('',(0.,0.,-1.));
#5913=DIRECTION('center_axis',(0.,1.,0.));
#5914=DIRECTION('ref_axis',(-0.896854406292881,0.,-0.442325868464691));
#5915=DIRECTION('center_axis',(0.,-1.,0.));
#5916=DIRECTION('ref_axis',(-0.896854406292881,0.,-0.442325868464691));
#5917=DIRECTION('',(-0.430412823330935,0.707106781186551,-0.561021213067998));
#5918=DIRECTION('center_axis',(0.,1.,0.));
#5919=DIRECTION('ref_axis',(-0.896854406292881,0.,-0.442325868464691));
#5920=DIRECTION('center_axis',(0.,-1.,0.));
#5921=DIRECTION('ref_axis',(-1.83697019872103E-16,0.,-1.));
#5922=DIRECTION('',(0.430412823330939,0.707106781186545,-0.561021213068002));
#5923=DIRECTION('center_axis',(0.,-1.,0.));
#5924=DIRECTION('ref_axis',(1.,0.,0.));
#5925=DIRECTION('center_axis',(0.,1.,0.));
#5926=DIRECTION('ref_axis',(1.,0.,0.));
#5927=DIRECTION('center_axis',(0.,1.,0.));
#5928=DIRECTION('ref_axis',(0.896854406292881,0.,-0.442325868464691));
#5929=DIRECTION('center_axis',(0.,-1.,0.));
#5930=DIRECTION('ref_axis',(0.896854406292881,0.,-0.442325868464691));
#5931=DIRECTION('',(0.707106781186547,0.707106781186547,0.));
#5932=DIRECTION('center_axis',(0.,1.,0.));
#5933=DIRECTION('ref_axis',(0.896854406292881,0.,-0.442325868464691));
#5934=DIRECTION('center_axis',(-0.707106781186546,0.707106781186549,0.));
#5935=DIRECTION('ref_axis',(0.,0.,1.));
#5936=DIRECTION('',(0.707106781186548,0.707106781186547,0.));
#5937=DIRECTION('',(0.,0.,-1.));
#5938=DIRECTION('',(0.,0.,1.));
#5939=DIRECTION('center_axis',(0.,1.,0.));
#5940=DIRECTION('ref_axis',(0.707106781186548,0.,0.707106781186548));
#5941=DIRECTION('center_axis',(0.,-1.,0.));
#5942=DIRECTION('ref_axis',(0.707106781186548,0.,0.707106781186548));
#5943=DIRECTION('',(0.,0.707106781186552,0.707106781186543));
#5944=DIRECTION('center_axis',(0.,1.,0.));
#5945=DIRECTION('ref_axis',(0.707106781186547,0.,0.707106781186547));
#5946=DIRECTION('center_axis',(0.,0.707106781186548,-0.707106781186548));
#5947=DIRECTION('ref_axis',(-1.,0.,0.));
#5948=DIRECTION('',(0.,0.707106781186547,0.707106781186547));
#5949=DIRECTION('',(1.,0.,0.));
#5950=DIRECTION('',(-1.,0.,0.));
#5951=DIRECTION('center_axis',(0.,0.,1.));
#5952=DIRECTION('ref_axis',(-1.,0.,0.));
#5953=DIRECTION('',(0.,-0.707106781186547,0.707106781186548));
#5954=DIRECTION('center_axis',(0.,0.,-1.));
#5955=DIRECTION('ref_axis',(-1.,0.,0.));
#5956=DIRECTION('center_axis',(0.,0.,1.));
#5957=DIRECTION('ref_axis',(-1.,0.,0.));
#5958=DIRECTION('center_axis',(0.,-0.707106781186548,-0.707106781186548));
#5959=DIRECTION('ref_axis',(-1.,0.,0.));
#5960=DIRECTION('',(0.,-0.707106781186547,0.707106781186547));
#5961=DIRECTION('',(-1.,0.,0.));
#5962=DIRECTION('',(1.,0.,0.));
#5963=DIRECTION('center_axis',(0.,-1.,0.));
#5964=DIRECTION('ref_axis',(0.707106781186548,0.,0.707106781186548));
#5965=DIRECTION('center_axis',(0.,1.,0.));
#5966=DIRECTION('ref_axis',(0.707106781186548,0.,0.707106781186548));
#5967=DIRECTION('',(0.707106781186547,-0.707106781186547,0.));
#5968=DIRECTION('center_axis',(0.,-1.,0.));
#5969=DIRECTION('ref_axis',(0.707106781186547,0.,0.707106781186547));
#5970=DIRECTION('center_axis',(-0.707106781186548,-0.707106781186548,0.));
#5971=DIRECTION('ref_axis',(0.,0.,1.));
#5972=DIRECTION('',(0.,0.,-1.));
#5973=DIRECTION('',(0.707106781186547,-0.707106781186547,0.));
#5974=DIRECTION('',(0.,0.,1.));
#5975=DIRECTION('center_axis',(0.,-1.,0.));
#5976=DIRECTION('ref_axis',(0.896854406292881,0.,-0.442325868464691));
#5977=DIRECTION('center_axis',(0.,1.,0.));
#5978=DIRECTION('ref_axis',(0.896854406292881,0.,-0.442325868464691));
#5979=DIRECTION('',(0.430412823330944,-0.707106781186546,-0.561021213067997));
#5980=DIRECTION('center_axis',(0.,-1.,0.));
#5981=DIRECTION('ref_axis',(0.896854406292881,0.,-0.442325868464691));
#5982=DIRECTION('center_axis',(0.,1.,0.));
#5983=DIRECTION('ref_axis',(-1.83697019872103E-16,0.,-1.));
#5984=DIRECTION('center_axis',(0.,-1.,0.));
#5985=DIRECTION('ref_axis',(1.,0.,0.));
#5986=DIRECTION('',(-0.430412823330944,-0.707106781186546,-0.561021213067997));
#5987=DIRECTION('center_axis',(0.,1.,0.));
#5988=DIRECTION('ref_axis',(1.,0.,0.));
#5989=DIRECTION('center_axis',(0.,-1.,0.));
#5990=DIRECTION('ref_axis',(-0.896854406292881,0.,-0.442325868464691));
#5991=DIRECTION('center_axis',(0.,1.,0.));
#5992=DIRECTION('ref_axis',(-0.896854406292881,0.,-0.442325868464691));
#5993=DIRECTION('center_axis',(0.,-1.,0.));
#5994=DIRECTION('ref_axis',(-0.896854406292881,0.,-0.442325868464691));
#5995=DIRECTION('center_axis',(0.,0.,1.));
#5996=DIRECTION('ref_axis',(1.,0.,0.));
#5997=DIRECTION('',(0.,-1.,0.));
#5998=DIRECTION('center_axis',(0.,0.,-1.));
#5999=DIRECTION('ref_axis',(1.,0.,0.));
#6000=DIRECTION('center_axis',(0.,1.,0.));
#6001=DIRECTION('ref_axis',(0.896854406292881,0.,-0.442325868464691));
#6002=DIRECTION('',(0.,-1.,0.));
#6003=DIRECTION('',(0.,1.,0.));
#6004=DIRECTION('center_axis',(0.,1.,0.));
#6005=DIRECTION('ref_axis',(5.0532154980743E-16,0.,-1.));
#6006=DIRECTION('',(0.,1.,0.));
#6007=DIRECTION('center_axis',(0.,1.,0.));
#6008=DIRECTION('ref_axis',(0.707106781186548,0.,0.707106781186548));
#6009=DIRECTION('',(0.,1.,0.));
#6010=DIRECTION('center_axis',(0.,1.,0.));
#6011=DIRECTION('ref_axis',(-0.896854406292882,0.,-0.442325868464691));
#6012=DIRECTION('',(0.,-1.,0.));
#6013=DIRECTION('center_axis',(1.,0.,0.));
#6014=DIRECTION('ref_axis',(0.,1.,0.));
#6015=DIRECTION('center_axis',(0.,-1.,0.));
#6016=DIRECTION('ref_axis',(1.,0.,0.));
#6017=DIRECTION('',(0.,0.,1.));
#6018=DIRECTION('center_axis',(0.,1.,0.));
#6019=DIRECTION('ref_axis',(1.,0.,0.));
#6020=DIRECTION('center_axis',(0.,0.,1.));
#6021=DIRECTION('ref_axis',(-1.,1.22464679914735E-16,0.));
#6022=DIRECTION('',(0.,0.,1.));
#6023=DIRECTION('center_axis',(-1.,0.,0.));
#6024=DIRECTION('ref_axis',(0.,0.,1.));
#6025=DIRECTION('',(0.,-1.,0.));
#6026=DIRECTION('center_axis',(0.,-1.,0.));
#6027=DIRECTION('ref_axis',(0.707106781186548,0.,0.707106781186548));
#6028=DIRECTION('',(0.,1.,0.));
#6029=DIRECTION('center_axis',(0.,1.,0.));
#6030=DIRECTION('ref_axis',(1.,0.,0.));
#6031=DIRECTION('',(0.,1.,0.));
#6032=DIRECTION('center_axis',(0.,-1.,0.));
#6033=DIRECTION('ref_axis',(1.,0.,0.));
#6034=DIRECTION('center_axis',(0.,0.,-1.));
#6035=DIRECTION('ref_axis',(1.,0.,0.));
#6036=DIRECTION('',(0.,0.,-1.));
#6037=DIRECTION('center_axis',(0.,0.,1.));
#6038=DIRECTION('ref_axis',(1.,0.,0.));
#6039=DIRECTION('center_axis',(0.,1.,0.));
#6040=DIRECTION('ref_axis',(-1.,0.,0.));
#6041=DIRECTION('center_axis',(0.,0.,1.));
#6042=DIRECTION('ref_axis',(1.,0.,0.));
#9215=CARTESIAN_POINT('',(0.,0.,0.));
#9216=CARTESIAN_POINT('Origin',(19.88,-2.88,7.));
#9217=CARTESIAN_POINT('',(20.,-2.76,8.6));
#9218=CARTESIAN_POINT('',(19.76,-3.,8.6));
#9219=CARTESIAN_POINT('',(20.,-2.76,8.6));
#9220=CARTESIAN_POINT('',(19.76,-3.,-2.35034248182107));
#9221=CARTESIAN_POINT('',(19.76,-3.,7.));
#9222=CARTESIAN_POINT('',(20.,-2.76,-2.35034248182107));
#9223=CARTESIAN_POINT('',(19.76,-3.,-2.35034248182107));
#9224=CARTESIAN_POINT('',(20.,-2.76,7.));
#9225=CARTESIAN_POINT('Origin',(19.2,-2.88,8.6));
#9226=CARTESIAN_POINT('',(19.2,-2.76,9.4));
#9227=CARTESIAN_POINT('Origin',(19.2,-2.76,8.6));
#9228=CARTESIAN_POINT('',(19.2,-3.,9.16));
#9229=CARTESIAN_POINT('',(19.2,-2.76,9.4));
#9230=CARTESIAN_POINT('Origin',(19.2,-3.,8.6));
#9231=CARTESIAN_POINT('Origin',(13.25,-2.88,9.28));
#9232=CARTESIAN_POINT('',(12.,-2.76,9.4));
#9233=CARTESIAN_POINT('',(13.25,-2.76,9.4));
#9234=CARTESIAN_POINT('',(12.,-3.,9.16));
#9235=CARTESIAN_POINT('',(12.,-2.76,9.4));
#9236=CARTESIAN_POINT('',(13.25,-3.,9.16));
#9237=CARTESIAN_POINT('Origin',(12.,0.,9.28));
#9238=CARTESIAN_POINT('',(12.,2.76,9.4));
#9239=CARTESIAN_POINT('Origin',(12.,0.,9.4));
#9240=CARTESIAN_POINT('',(12.,3.,9.16));
#9241=CARTESIAN_POINT('',(12.,2.76,9.4));
#9242=CARTESIAN_POINT('Origin',(12.,0.,9.16));
#9243=CARTESIAN_POINT('Origin',(17.25,2.88,9.28));
#9244=CARTESIAN_POINT('',(19.2,2.76,9.4));
#9245=CARTESIAN_POINT('',(17.25,2.76,9.4));
#9246=CARTESIAN_POINT('',(19.2,3.,9.16));
#9247=CARTESIAN_POINT('',(19.2,2.76,9.4));
#9248=CARTESIAN_POINT('',(17.25,3.,9.16));
#9249=CARTESIAN_POINT('Origin',(19.2,2.88,8.6));
#9250=CARTESIAN_POINT('',(20.,2.76,8.6));
#9251=CARTESIAN_POINT('Origin',(19.2,2.76,8.6));
#9252=CARTESIAN_POINT('',(19.76,3.,8.6));
#9253=CARTESIAN_POINT('',(20.,2.76,8.6));
#9254=CARTESIAN_POINT('Origin',(19.2,3.,8.6));
#9255=CARTESIAN_POINT('Origin',(19.88,2.88,7.));
#9256=CARTESIAN_POINT('',(20.,2.76,-2.35034248182107));
#9257=CARTESIAN_POINT('',(19.76,3.,-2.35034248182107));
#9258=CARTESIAN_POINT('',(20.,2.76,-2.35034248182107));
#9259=CARTESIAN_POINT('',(19.76,3.,7.));
#9260=CARTESIAN_POINT('',(20.,2.76,7.));
#9261=CARTESIAN_POINT('Origin',(20.8,2.88,-2.35034248182107));
#9262=CARTESIAN_POINT('',(20.3130434782609,2.76,-2.98506552846088));
#9263=CARTESIAN_POINT('Origin',(20.8,2.76,-2.35034248182107));
#9264=CARTESIAN_POINT('',(20.1669565217391,3.,-3.17548244245282));
#9265=CARTESIAN_POINT('',(20.3130434782609,2.76,-2.98506552846088));
#9266=CARTESIAN_POINT('Origin',(20.8,3.,-2.35034248182107));
#9267=CARTESIAN_POINT('Origin',(18.,2.88,-6.));
#9268=CARTESIAN_POINT('',(15.6869565217391,2.76,-2.98506552846088));
#9269=CARTESIAN_POINT('',(15.8330434782609,3.,-3.17548244245283));
#9270=CARTESIAN_POINT('',(15.6869565217391,2.76,-2.98506552846088));
#9271=CARTESIAN_POINT('Origin',(18.,3.,-6.));
#9272=CARTESIAN_POINT('Origin',(18.,2.76,-6.));
#9273=CARTESIAN_POINT('Origin',(15.2,2.88,-2.35034248182107));
#9274=CARTESIAN_POINT('',(16.,2.76,-2.35034248182107));
#9275=CARTESIAN_POINT('Origin',(15.2,2.76,-2.35034248182107));
#9276=CARTESIAN_POINT('',(16.24,3.,-2.35034248182107));
#9277=CARTESIAN_POINT('',(16.,2.76,-2.35034248182107));
#9278=CARTESIAN_POINT('Origin',(15.2,3.,-2.35034248182107));
#9279=CARTESIAN_POINT('Origin',(16.12,2.88,2.11554944214035));
#9280=CARTESIAN_POINT('',(16.,2.76,6.2));
#9281=CARTESIAN_POINT('',(16.24,3.,6.2));
#9282=CARTESIAN_POINT('',(16.,2.76,6.2));
#9283=CARTESIAN_POINT('',(16.24,3.,2.11554944214035));
#9284=CARTESIAN_POINT('',(16.,2.76,2.11554944214035));
#9285=CARTESIAN_POINT('Origin',(15.2,2.88,6.2));
#9286=CARTESIAN_POINT('',(15.2,2.76,7.));
#9287=CARTESIAN_POINT('Origin',(15.2,2.76,6.2));
#9288=CARTESIAN_POINT('',(15.2,3.,7.24));
#9289=CARTESIAN_POINT('',(15.2,2.76,7.));
#9290=CARTESIAN_POINT('Origin',(15.2,3.,6.2));
#9291=CARTESIAN_POINT('Origin',(17.25,2.88,7.12));
#9292=CARTESIAN_POINT('',(12.,2.76,7.));
#9293=CARTESIAN_POINT('',(12.,3.,7.24));
#9294=CARTESIAN_POINT('',(12.,2.76,7.));
#9295=CARTESIAN_POINT('',(17.25,3.,7.24));
#9296=CARTESIAN_POINT('',(17.25,2.76,7.));
#9297=CARTESIAN_POINT('Origin',(12.,0.,7.12));
#9298=CARTESIAN_POINT('',(12.,-2.76,7.));
#9299=CARTESIAN_POINT('',(12.,-3.,7.24));
#9300=CARTESIAN_POINT('',(12.,-2.76,7.));
#9301=CARTESIAN_POINT('Origin',(12.,0.,7.24));
#9302=CARTESIAN_POINT('Origin',(12.,0.,7.));
#9303=CARTESIAN_POINT('Origin',(13.25,-2.88,7.12));
#9304=CARTESIAN_POINT('',(15.2,-2.76,7.));
#9305=CARTESIAN_POINT('',(15.2,-3.,7.24));
#9306=CARTESIAN_POINT('',(15.2,-2.76,7.));
#9307=CARTESIAN_POINT('',(13.25,-3.,7.24));
#9308=CARTESIAN_POINT('',(13.25,-2.76,7.));
#9309=CARTESIAN_POINT('Origin',(15.2,-2.88,6.2));
#9310=CARTESIAN_POINT('',(16.,-2.76,6.2));
#9311=CARTESIAN_POINT('Origin',(15.2,-2.76,6.2));
#9312=CARTESIAN_POINT('',(16.24,-3.,6.2));
#9313=CARTESIAN_POINT('',(16.,-2.76,6.2));
#9314=CARTESIAN_POINT('Origin',(15.2,-3.,6.2));
#9315=CARTESIAN_POINT('Origin',(16.12,-2.88,2.11554944214035));
#9316=CARTESIAN_POINT('',(16.,-2.76,-2.35034248182107));
#9317=CARTESIAN_POINT('',(16.,-2.76,2.11554944214035));
#9318=CARTESIAN_POINT('',(16.24,-3.,-2.35034248182107));
#9319=CARTESIAN_POINT('',(16.,-2.76,-2.35034248182107));
#9320=CARTESIAN_POINT('',(16.24,-3.,2.11554944214035));
#9321=CARTESIAN_POINT('Origin',(15.2,-2.88,-2.35034248182107));
#9322=CARTESIAN_POINT('',(15.6869565217391,-2.76,-2.98506552846088));
#9323=CARTESIAN_POINT('Origin',(15.2,-2.76,-2.35034248182107));
#9324=CARTESIAN_POINT('',(15.8330434782609,-3.,-3.17548244245283));
#9325=CARTESIAN_POINT('',(15.6869565217391,-2.76,-2.98506552846088));
#9326=CARTESIAN_POINT('Origin',(15.2,-3.,-2.35034248182107));
#9327=CARTESIAN_POINT('Origin',(18.,-2.88,-6.));
#9328=CARTESIAN_POINT('',(20.3130434782609,-2.76,-2.98506552846088));
#9329=CARTESIAN_POINT('Origin',(18.,-2.76,-6.));
#9330=CARTESIAN_POINT('',(20.1669565217391,-3.,-3.17548244245283));
#9331=CARTESIAN_POINT('',(20.3130434782609,-2.76,-2.98506552846088));
#9332=CARTESIAN_POINT('Origin',(18.,-3.,-6.));
#9333=CARTESIAN_POINT('Origin',(20.8,-2.88,-2.35034248182107));
#9334=CARTESIAN_POINT('Origin',(20.8,-2.76,-2.35034248182107));
#9335=CARTESIAN_POINT('Origin',(20.8,-3.,-2.35034248182107));
#9336=CARTESIAN_POINT('Origin',(14.5,0.,9.4));
#9337=CARTESIAN_POINT('',(19.2,-1.5,9.4));
#9338=CARTESIAN_POINT('',(10.95,-1.28587913910472E-16,9.4));
#9339=CARTESIAN_POINT('Origin',(12.,0.,9.4));
#9340=CARTESIAN_POINT('Origin',(15.2,-3.,-2.35034248182107));
#9341=CARTESIAN_POINT('',(15.6869565217391,-3.,-2.98506552846088));
#9342=CARTESIAN_POINT('',(16.,-3.,-2.35034248182107));
#9343=CARTESIAN_POINT('Origin',(18.,-3.,-6.));
#9344=CARTESIAN_POINT('',(20.3130434782609,-3.,-2.98506552846088));
#9345=CARTESIAN_POINT('Origin',(19.2,-1.5,8.6));
#9346=CARTESIAN_POINT('',(20.,-1.5,8.6));
#9347=CARTESIAN_POINT('Origin',(20.8,-3.,-2.35034248182107));
#9348=CARTESIAN_POINT('',(20.,-3.,-2.35034248182107));
#9349=CARTESIAN_POINT('Origin',(20.,-3.,7.));
#9350=CARTESIAN_POINT('Origin',(12.,-3.,7.));
#9351=CARTESIAN_POINT('',(12.,-3.,7.));
#9352=CARTESIAN_POINT('',(15.99,-3.,-6.));
#9353=CARTESIAN_POINT('Origin',(18.,-3.,-6.));
#9354=CARTESIAN_POINT('Origin',(12.,0.,7.));
#9355=CARTESIAN_POINT('',(12.,3.,7.));
#9356=CARTESIAN_POINT('Origin',(16.,-3.,-2.7689011157193));
#9357=CARTESIAN_POINT('',(16.,-1.5,6.2));
#9358=CARTESIAN_POINT('Origin',(15.2,-1.5,6.2));
#9359=CARTESIAN_POINT('',(15.2,-1.5,7.));
#9360=CARTESIAN_POINT('Origin',(18.,-3.,-6.));
#9361=CARTESIAN_POINT('',(15.99,3.,-6.));
#9362=CARTESIAN_POINT('',(15.99,-3.,-6.));
#9363=CARTESIAN_POINT('Origin',(18.,3.,-6.));
#9364=CARTESIAN_POINT('Origin',(12.,0.,9.4));
#9365=CARTESIAN_POINT('',(10.95,-1.28587913910472E-16,7.));
#9366=CARTESIAN_POINT('',(10.95,1.28587913910472E-16,9.4));
#9367=CARTESIAN_POINT('Origin',(12.,0.,7.));
#9368=CARTESIAN_POINT('Origin',(20.,3.,7.));
#9369=CARTESIAN_POINT('Origin',(14.5,0.,7.));
#11412=UNCERTAINTY_MEASURE_WITH_UNIT(LENGTH_MEASURE(0.01),#11431,
'DISTANCE_ACCURACY_VALUE',
'Maximum model space distance between geometric entities at asserted c
onnectivities');
#11416=UNCERTAINTY_MEASURE_WITH_UNIT(LENGTH_MEASURE(0.01),#11431,
'DISTANCE_ACCURACY_VALUE',
'Maximum model space distance between geometric entities at asserted c
onnectivities');
#11426=(
GEOMETRIC_REPRESENTATION_CONTEXT(3)
GLOBAL_UNCERTAINTY_ASSIGNED_CONTEXT((#11412))
GLOBAL_UNIT_ASSIGNED_CONTEXT((#11431,#11433,#11434))
REPRESENTATION_CONTEXT('','3D')
);
#11430=(
GEOMETRIC_REPRESENTATION_CONTEXT(3)
GLOBAL_UNCERTAINTY_ASSIGNED_CONTEXT((#11416))
GLOBAL_UNIT_ASSIGNED_CONTEXT((#11431,#11433,#11434))
REPRESENTATION_CONTEXT('','3D')
);
#11431=(
LENGTH_UNIT()
NAMED_UNIT(*)
SI_UNIT(.MILLI.,.METRE.)
);
#11433=(
NAMED_UNIT(*)
PLANE_ANGLE_UNIT()
SI_UNIT($,.RADIAN.)
);
#11434=(
NAMED_UNIT(*)
SI_UNIT($,.STERADIAN.)
SOLID_ANGLE_UNIT()
);
#11444=SHAPE_DEFINITION_REPRESENTATION(#11457,#11487);
#11457=PRODUCT_DEFINITION_SHAPE('',$,#11501);
#11487=SHAPE_REPRESENTATION('',(#4914),#11426);
#11491=PRODUCT_DEFINITION_CONTEXT('part definition',#11532,'design');
#11501=PRODUCT_DEFINITION('2026-10-25-00-55-38-878',
'07_Pitch_Link_Black',#11514,#11491);
#11514=PRODUCT_DEFINITION_FORMATION('',$,#11543);
#11532=APPLICATION_CONTEXT(
'Core Data for Automotive Mechanical Design Process');
#11533=PRODUCT_CONTEXT('part definition',#11532,'mechanical');
#11543=PRODUCT('2026-10-25-00-55-38-878','07_Pitch_Link_Black',$,(#11533));
#11617=COLOUR_RGB('Off White',0.89,0.88,0.83);
#11618=FILL_AREA_STYLE_COLOUR('',#11617);
#11619=FILL_AREA_STYLE('',(#11618));
#11620=SURFACE_STYLE_FILL_AREA(#11619);
#11621=SURFACE_SIDE_STYLE('',(#11620));
#11622=SURFACE_STYLE_USAGE(.BOTH.,#11621);
#11623=PRESENTATION_STYLE_ASSIGNMENT((#11622));
ENDSEC;
END-ISO-10303-21;
